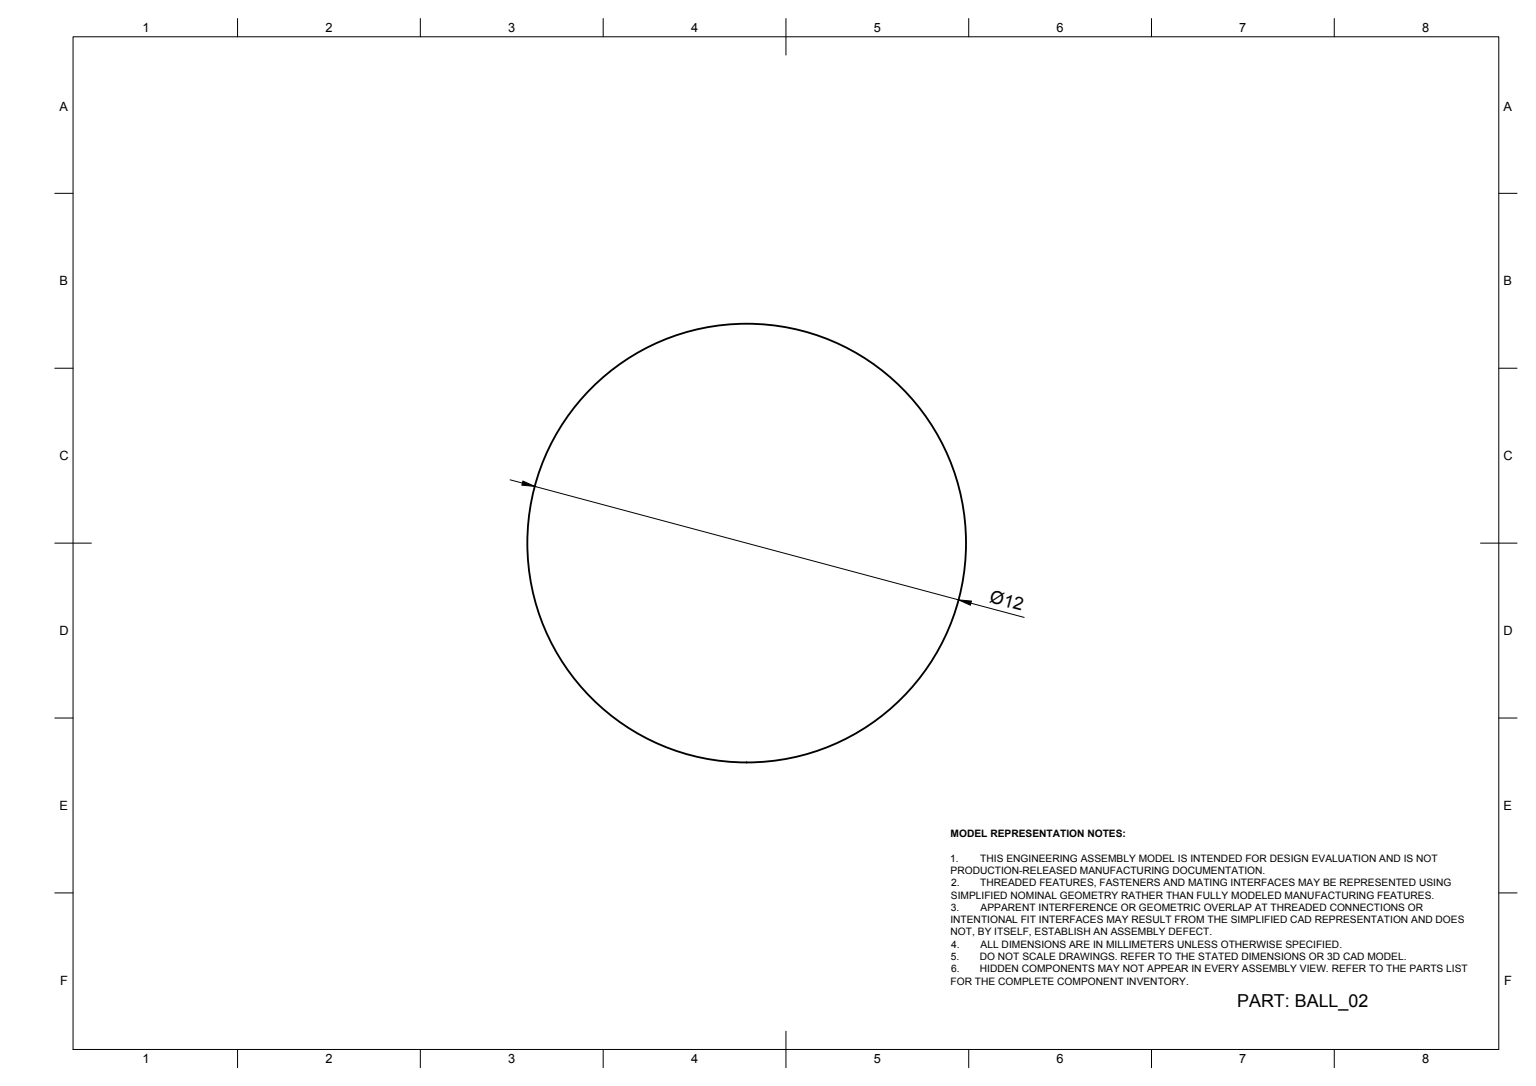
ISO-10303-21;
HEADER;
/* Generated by software containing ST-Developer
 * from STEP Tools, Inc. (www.steptools.com) 
 */

FILE_DESCRIPTION(
/* description */ (''),
/* implementation_level */ '2;1');

FILE_NAME(
/* name */ 'Ball_02.step',
/* time_stamp */ '2026-10-05T00:14:20-07:00',
/* author */ (''),
/* organization */ (''),
/* preprocessor_version */ 'ST-DEVELOPER v20.2',
/* originating_system */ 'Autodesk Translation Framework v15.15.0.0',
/* authorisation */ '');

FILE_SCHEMA (('AUTOMOTIVE_DESIGN { 1 0 10303 214 3 1 1 }'));
ENDSEC;

DATA;
#10=MECHANICAL_DESIGN_GEOMETRIC_PRESENTATION_REPRESENTATION('',(#3373),#75336);
#3353=SPHERICAL_SURFACE('',#32138,6.);
#3357=SHAPE_REPRESENTATION_RELATIONSHIP('SRR','None',#75370,#3365);
#3365=ADVANCED_BREP_SHAPE_REPRESENTATION('',(#3381),#75330);
#3373=STYLED_ITEM('',(#75418),#3381);
#3381=MANIFOLD_SOLID_BREP('Body1',#32023);
#3403=CIRCLE('',#32139,6.);
#5147=FACE_OUTER_BOUND('',#6875,.T.);
#6875=EDGE_LOOP('',(#19627,#19628));
#11110=VERTEX_POINT('',#46105);
#11111=VERTEX_POINT('',#46106);
#14508=EDGE_CURVE('',#11110,#11111,#3403,.T.);
#19627=ORIENTED_EDGE('',*,*,#14508,.T.);
#19628=ORIENTED_EDGE('',*,*,#14508,.F.);
#30307=ADVANCED_FACE('',(#5147),#3353,.T.);
#32023=CLOSED_SHELL('',(#30307));
#32137=AXIS2_PLACEMENT_3D('',#46103,#36405,#36406);
#32138=AXIS2_PLACEMENT_3D('',#46104,#36407,#36408);
#32139=AXIS2_PLACEMENT_3D('',#46107,#36409,#36410);
#36405=DIRECTION('axis',(0.,0.,1.));
#36406=DIRECTION('refdir',(1.,0.,0.));
#36407=DIRECTION('center_axis',(0.,0.,1.));
#36408=DIRECTION('ref_axis',(-0.5,0.866025403784439,0.));
#36409=DIRECTION('center_axis',(0.866025403784439,0.5,0.));
#36410=DIRECTION('ref_axis',(0.5,-0.866025403784439,0.));
#46103=CARTESIAN_POINT('',(0.,0.,0.));
#46104=CARTESIAN_POINT('Origin',(-15.,25.9807621135332,13.));
#46105=CARTESIAN_POINT('',(-15.,25.9807621135332,19.));
#46106=CARTESIAN_POINT('',(-15.,25.9807621135332,7.));
#46107=CARTESIAN_POINT('Origin',(-15.,25.9807621135332,13.));
#75320=UNCERTAINTY_MEASURE_WITH_UNIT(LENGTH_MEASURE(0.01),#75337,
'DISTANCE_ACCURACY_VALUE',
'Maximum model space distance between geometric entities at asserted c
onnectivities');
#75326=UNCERTAINTY_MEASURE_WITH_UNIT(LENGTH_MEASURE(0.01),#75337,
'DISTANCE_ACCURACY_VALUE',
'Maximum model space distance between geometric entities at asserted c
onnectivities');
#75330=(
GEOMETRIC_REPRESENTATION_CONTEXT(3)
GLOBAL_UNCERTAINTY_ASSIGNED_CONTEXT((#75320))
GLOBAL_UNIT_ASSIGNED_CONTEXT((#75337,#75339,#75340))
REPRESENTATION_CONTEXT('','3D')
);
#75336=(
GEOMETRIC_REPRESENTATION_CONTEXT(3)
GLOBAL_UNCERTAINTY_ASSIGNED_CONTEXT((#75326))
GLOBAL_UNIT_ASSIGNED_CONTEXT((#75337,#75339,#75340))
REPRESENTATION_CONTEXT('','3D')
);
#75337=(
LENGTH_UNIT()
NAMED_UNIT(*)
SI_UNIT(.MILLI.,.METRE.)
);
#75339=(
NAMED_UNIT(*)
PLANE_ANGLE_UNIT()
SI_UNIT($,.RADIAN.)
);
#75340=(
NAMED_UNIT(*)
SI_UNIT($,.STERADIAN.)
SOLID_ANGLE_UNIT()
);
#75344=SHAPE_DEFINITION_REPRESENTATION(#75353,#75370);
#75353=PRODUCT_DEFINITION_SHAPE('',$,#75380);
#75370=SHAPE_REPRESENTATION('',(#32137),#75330);
#75376=PRODUCT_DEFINITION_CONTEXT('part definition',#75405,'design');
#75380=PRODUCT_DEFINITION('Ball_02','Ball_02',#75389,#75376);
#75389=PRODUCT_DEFINITION_FORMATION('',$,#75410);
#75405=APPLICATION_CONTEXT(
'Core Data for Automotive Mechanical Design Process');
#75406=PRODUCT_CONTEXT('part definition',#75405,'mechanical');
#75410=PRODUCT('Ball_02','Ball_02',$,(#75406));
#75418=PRESENTATION_STYLE_ASSIGNMENT((#75422));
#75422=SURFACE_STYLE_USAGE(.BOTH.,#75426);
#75426=SURFACE_SIDE_STYLE('',(#75430));
#75430=SURFACE_STYLE_FILL_AREA(#75434);
#75434=FILL_AREA_STYLE('Opaque(200,203,41)',(#75438));
#75438=FILL_AREA_STYLE_COLOUR('Opaque(200,203,41)',#75442);
#75442=COLOUR_RGB('Opaque(200,203,41)', 0.66274510, 0.83137255, 0.94901961);
ENDSEC;
END-ISO-10303-21;
